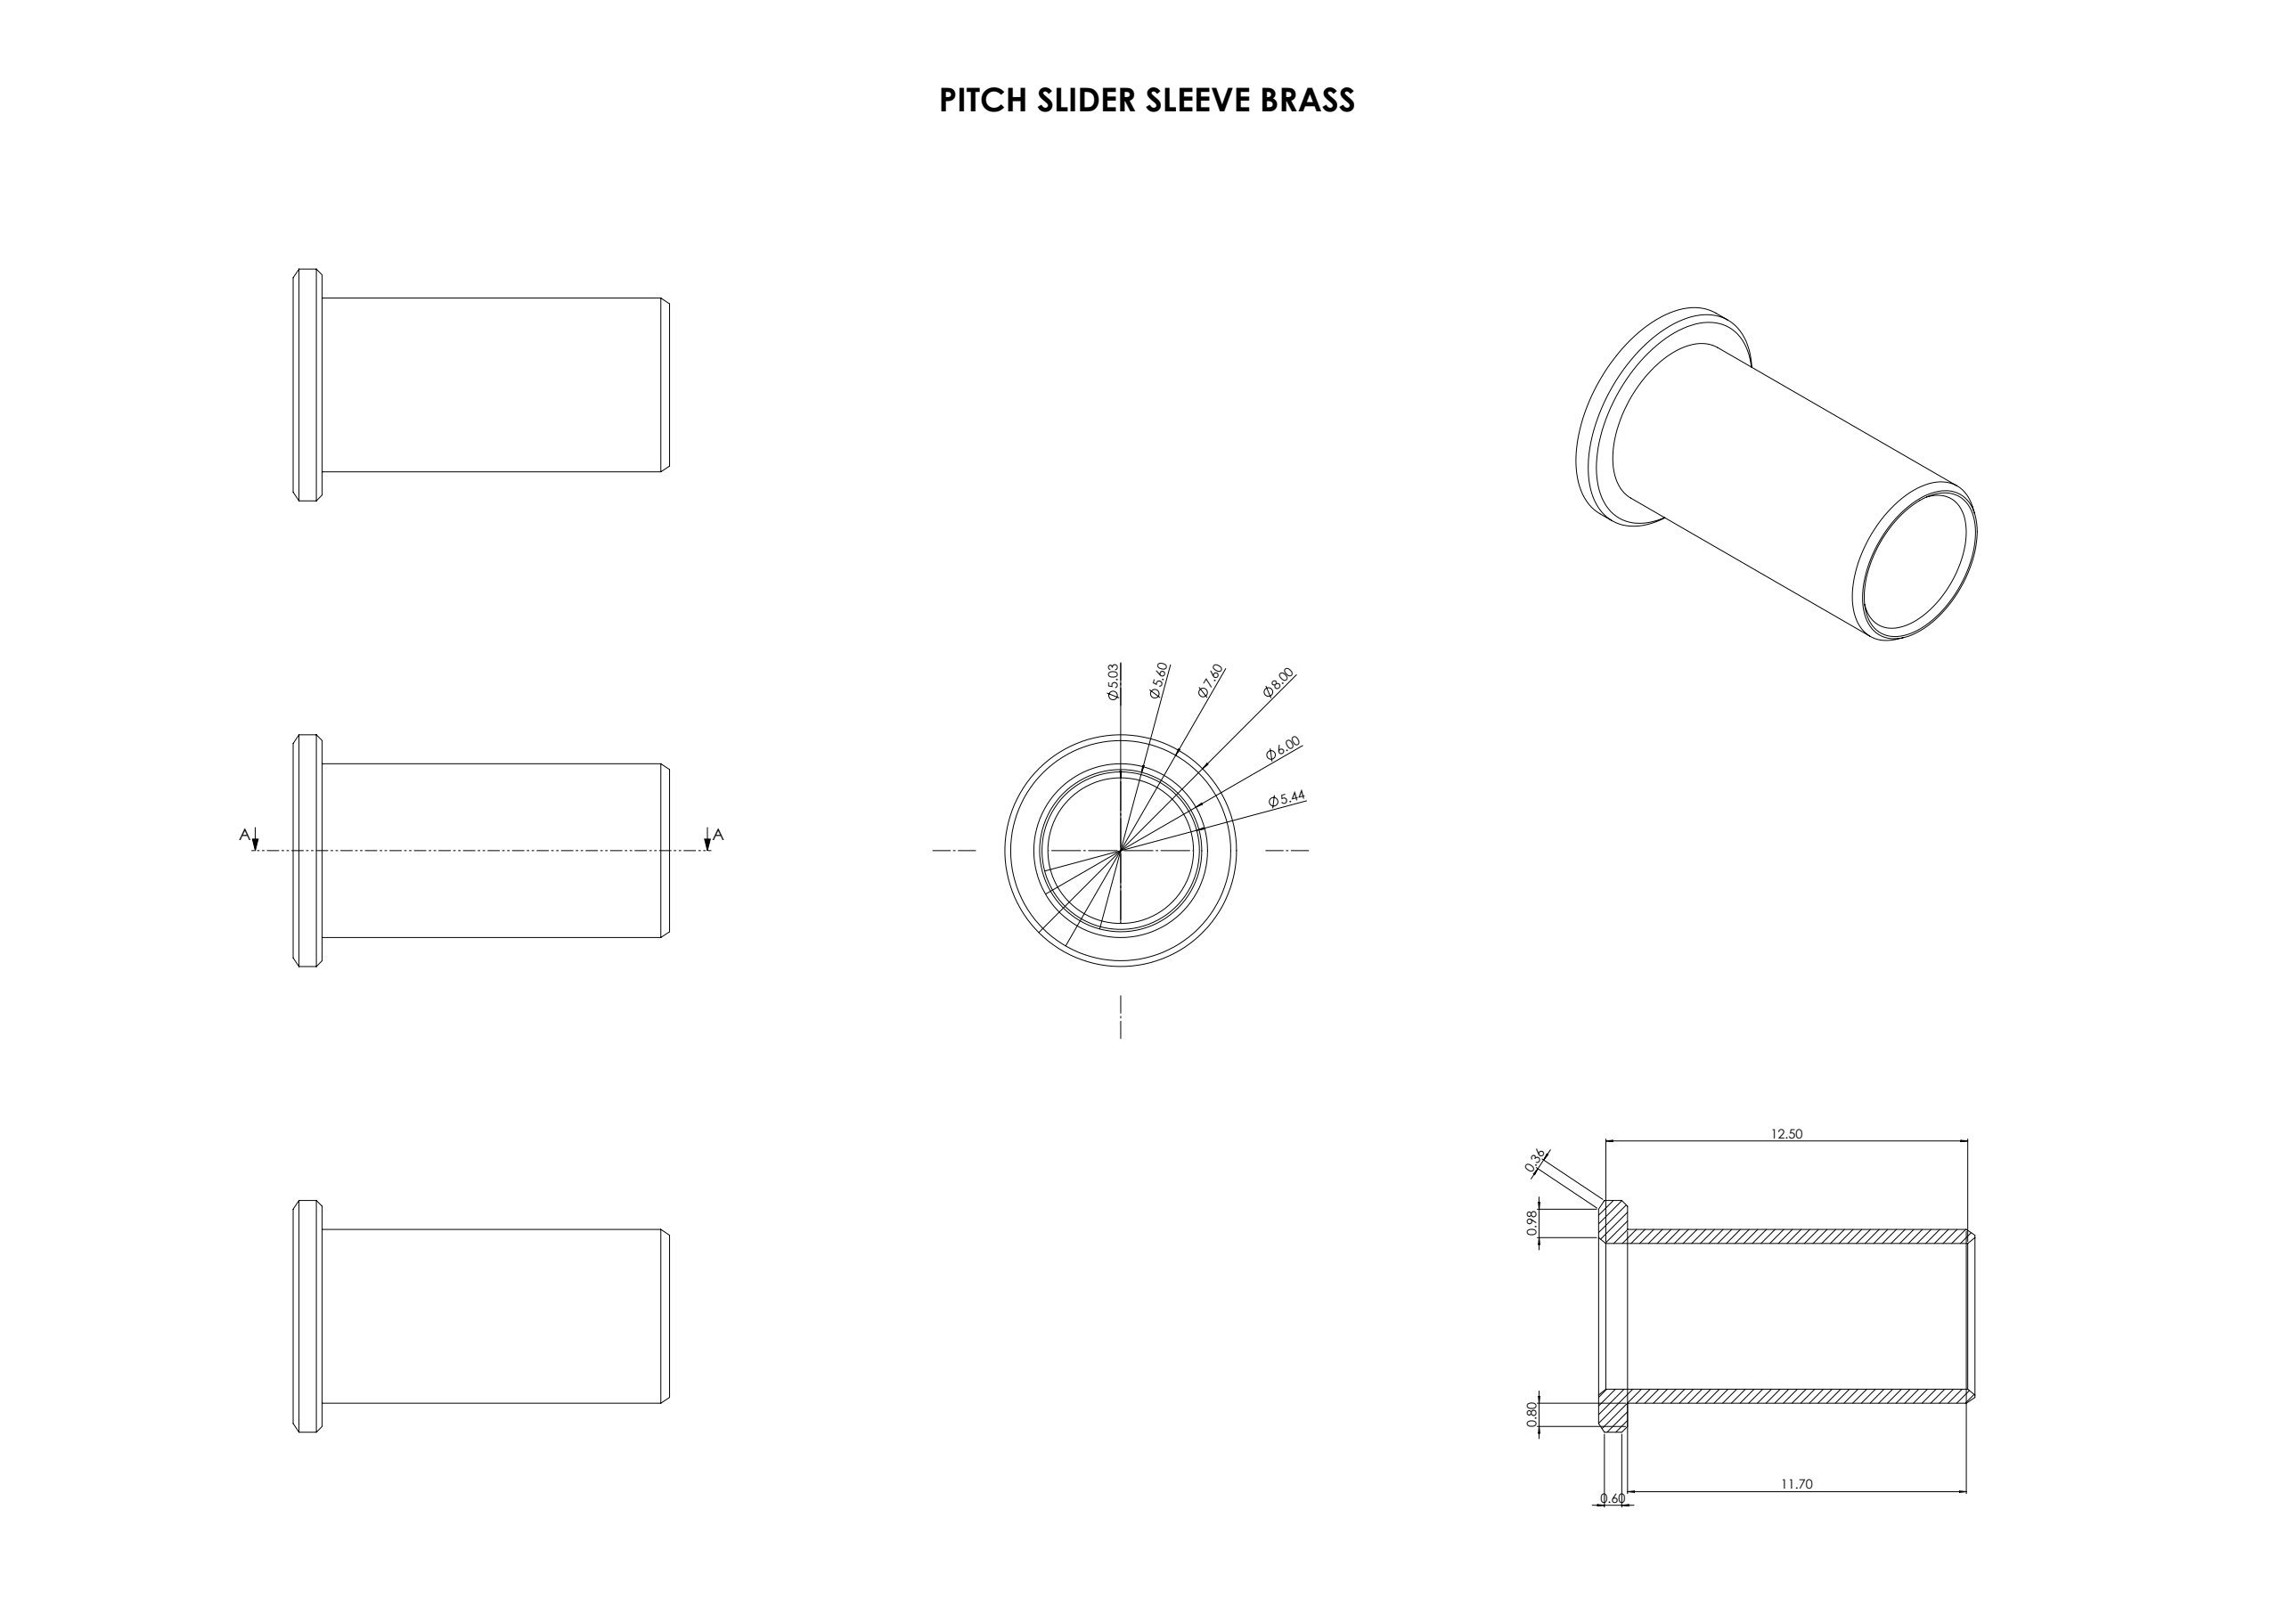
ISO-10303-21;
HEADER;
/* Generated by software containing ST-Developer
 * from STEP Tools, Inc. (www.steptools.com) 
 */

FILE_DESCRIPTION(
/* description */ (''),
/* implementation_level */ '2;1');

FILE_NAME(
/* name */ '02_Pitch_Slider_Sleeve_Brass.step',
/* time_stamp */ '2026-10-25T01:35:35-07:00',
/* author */ (''),
/* organization */ (''),
/* preprocessor_version */ 'ST-DEVELOPER v20.2',
/* originating_system */ 'Autodesk Translation Framework v15.15.0.0',
/* authorisation */ '');

FILE_SCHEMA (('AUTOMOTIVE_DESIGN { 1 0 10303 214 3 1 1 }'));
ENDSEC;

DATA;
#10=MECHANICAL_DESIGN_GEOMETRIC_PRESENTATION_REPRESENTATION('',(#261),#11430);
#237=SHAPE_REPRESENTATION_RELATIONSHIP('SRR','None',#11480,#249);
#249=ADVANCED_BREP_SHAPE_REPRESENTATION('',(#273),#11419);
#261=STYLED_ITEM('',(#11602),#273);
#273=MANIFOLD_SOLID_BREP('Body1',#4462);
#289=FACE_BOUND('',#842,.T.);
#290=FACE_BOUND('',#847,.T.);
#291=FACE_BOUND('',#851,.T.);
#342=PLANE('',#4685);
#343=PLANE('',#4693);
#344=PLANE('',#4699);
#440=CYLINDRICAL_SURFACE('',#4684,2.515);
#441=CYLINDRICAL_SURFACE('',#4689,4.);
#442=CYLINDRICAL_SURFACE('',#4695,3.);
#565=FACE_OUTER_BOUND('',#838,.T.);
#566=FACE_OUTER_BOUND('',#839,.T.);
#567=FACE_OUTER_BOUND('',#840,.T.);
#568=FACE_OUTER_BOUND('',#841,.T.);
#569=FACE_OUTER_BOUND('',#843,.T.);
#570=FACE_OUTER_BOUND('',#844,.T.);
#571=FACE_OUTER_BOUND('',#845,.T.);
#572=FACE_OUTER_BOUND('',#846,.T.);
#573=FACE_OUTER_BOUND('',#848,.T.);
#574=FACE_OUTER_BOUND('',#849,.T.);
#575=FACE_OUTER_BOUND('',#850,.T.);
#838=EDGE_LOOP('',(#3045,#3046,#3047,#3048));
#839=EDGE_LOOP('',(#3049,#3050,#3051,#3052));
#840=EDGE_LOOP('',(#3053,#3054,#3055,#3056));
#841=EDGE_LOOP('',(#3057));
#842=EDGE_LOOP('',(#3058));
#843=EDGE_LOOP('',(#3059,#3060,#3061,#3062));
#844=EDGE_LOOP('',(#3063,#3064,#3065,#3066));
#845=EDGE_LOOP('',(#3067,#3068,#3069,#3070));
#846=EDGE_LOOP('',(#3071));
#847=EDGE_LOOP('',(#3072));
#848=EDGE_LOOP('',(#3073,#3074,#3075,#3076));
#849=EDGE_LOOP('',(#3077,#3078,#3079,#3080));
#850=EDGE_LOOP('',(#3081));
#851=EDGE_LOOP('',(#3082));
#1151=LINE('',#6499,#1441);
#1152=LINE('',#6505,#1442);
#1153=LINE('',#6508,#1443);
#1154=LINE('',#6515,#1444);
#1155=LINE('',#6519,#1445);
#1156=LINE('',#6523,#1446);
#1157=LINE('',#6530,#1447);
#1158=LINE('',#6534,#1448);
#1441=VECTOR('',#5281,2.6575);
#1442=VECTOR('',#5288,2.6575);
#1443=VECTOR('',#5293,2.515);
#1444=VECTOR('',#5302,3.85);
#1445=VECTOR('',#5307,4.);
#1446=VECTOR('',#5312,3.9);
#1447=VECTOR('',#5321,3.);
#1448=VECTOR('',#5326,2.9);
#1711=CIRCLE('',#4679,2.515);
#1712=CIRCLE('',#4680,2.71857142857143);
#1713=CIRCLE('',#4682,2.71857142857143);
#1714=CIRCLE('',#4683,2.515);
#1715=CIRCLE('',#4686,3.7);
#1716=CIRCLE('',#4688,4.);
#1717=CIRCLE('',#4690,4.);
#1718=CIRCLE('',#4692,3.8);
#1719=CIRCLE('',#4694,3.);
#1720=CIRCLE('',#4696,3.);
#1721=CIRCLE('',#4698,2.8);
#1912=VERTEX_POINT('',#6496);
#1913=VERTEX_POINT('',#6498);
#1914=VERTEX_POINT('',#6502);
#1915=VERTEX_POINT('',#6504);
#1916=VERTEX_POINT('',#6510);
#1917=VERTEX_POINT('',#6513);
#1918=VERTEX_POINT('',#6517);
#1919=VERTEX_POINT('',#6521);
#1920=VERTEX_POINT('',#6525);
#1921=VERTEX_POINT('',#6528);
#1922=VERTEX_POINT('',#6532);
#2340=EDGE_CURVE('',#1912,#1912,#1711,.T.);
#2341=EDGE_CURVE('',#1912,#1913,#1151,.T.);
#2342=EDGE_CURVE('',#1913,#1913,#1712,.T.);
#2343=EDGE_CURVE('',#1914,#1914,#1713,.T.);
#2344=EDGE_CURVE('',#1914,#1915,#1152,.T.);
#2345=EDGE_CURVE('',#1915,#1915,#1714,.T.);
#2346=EDGE_CURVE('',#1912,#1915,#1153,.T.);
#2347=EDGE_CURVE('',#1916,#1916,#1715,.T.);
#2348=EDGE_CURVE('',#1917,#1917,#1716,.T.);
#2349=EDGE_CURVE('',#1917,#1916,#1154,.T.);
#2350=EDGE_CURVE('',#1918,#1918,#1717,.T.);
#2351=EDGE_CURVE('',#1918,#1917,#1155,.T.);
#2352=EDGE_CURVE('',#1919,#1919,#1718,.T.);
#2353=EDGE_CURVE('',#1919,#1918,#1156,.T.);
#2354=EDGE_CURVE('',#1920,#1920,#1719,.T.);
#2355=EDGE_CURVE('',#1921,#1921,#1720,.T.);
#2356=EDGE_CURVE('',#1921,#1920,#1157,.T.);
#2357=EDGE_CURVE('',#1922,#1922,#1721,.T.);
#2358=EDGE_CURVE('',#1922,#1921,#1158,.T.);
#3045=ORIENTED_EDGE('',*,*,#2340,.F.);
#3046=ORIENTED_EDGE('',*,*,#2341,.T.);
#3047=ORIENTED_EDGE('',*,*,#2342,.F.);
#3048=ORIENTED_EDGE('',*,*,#2341,.F.);
#3049=ORIENTED_EDGE('',*,*,#2343,.F.);
#3050=ORIENTED_EDGE('',*,*,#2344,.T.);
#3051=ORIENTED_EDGE('',*,*,#2345,.F.);
#3052=ORIENTED_EDGE('',*,*,#2344,.F.);
#3053=ORIENTED_EDGE('',*,*,#2340,.T.);
#3054=ORIENTED_EDGE('',*,*,#2346,.T.);
#3055=ORIENTED_EDGE('',*,*,#2345,.T.);
#3056=ORIENTED_EDGE('',*,*,#2346,.F.);
#3057=ORIENTED_EDGE('',*,*,#2347,.F.);
#3058=ORIENTED_EDGE('',*,*,#2343,.T.);
#3059=ORIENTED_EDGE('',*,*,#2348,.F.);
#3060=ORIENTED_EDGE('',*,*,#2349,.T.);
#3061=ORIENTED_EDGE('',*,*,#2347,.T.);
#3062=ORIENTED_EDGE('',*,*,#2349,.F.);
#3063=ORIENTED_EDGE('',*,*,#2350,.F.);
#3064=ORIENTED_EDGE('',*,*,#2351,.T.);
#3065=ORIENTED_EDGE('',*,*,#2348,.T.);
#3066=ORIENTED_EDGE('',*,*,#2351,.F.);
#3067=ORIENTED_EDGE('',*,*,#2352,.F.);
#3068=ORIENTED_EDGE('',*,*,#2353,.T.);
#3069=ORIENTED_EDGE('',*,*,#2350,.T.);
#3070=ORIENTED_EDGE('',*,*,#2353,.F.);
#3071=ORIENTED_EDGE('',*,*,#2352,.T.);
#3072=ORIENTED_EDGE('',*,*,#2354,.F.);
#3073=ORIENTED_EDGE('',*,*,#2355,.F.);
#3074=ORIENTED_EDGE('',*,*,#2356,.T.);
#3075=ORIENTED_EDGE('',*,*,#2354,.T.);
#3076=ORIENTED_EDGE('',*,*,#2356,.F.);
#3077=ORIENTED_EDGE('',*,*,#2357,.F.);
#3078=ORIENTED_EDGE('',*,*,#2358,.T.);
#3079=ORIENTED_EDGE('',*,*,#2355,.T.);
#3080=ORIENTED_EDGE('',*,*,#2358,.F.);
#3081=ORIENTED_EDGE('',*,*,#2357,.T.);
#3082=ORIENTED_EDGE('',*,*,#2342,.T.);
#4146=CONICAL_SURFACE('',#4678,2.6575,0.683391245487337);
#4147=CONICAL_SURFACE('',#4681,2.6575,0.683391245487336);
#4148=CONICAL_SURFACE('',#4687,3.85,0.982793723247329);
#4149=CONICAL_SURFACE('',#4691,3.9,0.785398163397449);
#4150=CONICAL_SURFACE('',#4697,2.9,0.588002603547568);
#4232=ADVANCED_FACE('',(#565),#4146,.F.);
#4233=ADVANCED_FACE('',(#566),#4147,.F.);
#4234=ADVANCED_FACE('',(#567),#440,.F.);
#4235=ADVANCED_FACE('',(#568,#289),#342,.T.);
#4236=ADVANCED_FACE('',(#569),#4148,.T.);
#4237=ADVANCED_FACE('',(#570),#441,.T.);
#4238=ADVANCED_FACE('',(#571),#4149,.T.);
#4239=ADVANCED_FACE('',(#572,#290),#343,.T.);
#4240=ADVANCED_FACE('',(#573),#442,.T.);
#4241=ADVANCED_FACE('',(#574),#4150,.T.);
#4242=ADVANCED_FACE('',(#575,#291),#344,.T.);
#4462=CLOSED_SHELL('',(#4232,#4233,#4234,#4235,#4236,#4237,#4238,#4239,
#4240,#4241,#4242));
#4677=AXIS2_PLACEMENT_3D('',#6494,#5275,#5276);
#4678=AXIS2_PLACEMENT_3D('',#6495,#5277,#5278);
#4679=AXIS2_PLACEMENT_3D('',#6497,#5279,#5280);
#4680=AXIS2_PLACEMENT_3D('',#6500,#5282,#5283);
#4681=AXIS2_PLACEMENT_3D('',#6501,#5284,#5285);
#4682=AXIS2_PLACEMENT_3D('',#6503,#5286,#5287);
#4683=AXIS2_PLACEMENT_3D('',#6506,#5289,#5290);
#4684=AXIS2_PLACEMENT_3D('',#6507,#5291,#5292);
#4685=AXIS2_PLACEMENT_3D('',#6509,#5294,#5295);
#4686=AXIS2_PLACEMENT_3D('',#6511,#5296,#5297);
#4687=AXIS2_PLACEMENT_3D('',#6512,#5298,#5299);
#4688=AXIS2_PLACEMENT_3D('',#6514,#5300,#5301);
#4689=AXIS2_PLACEMENT_3D('',#6516,#5303,#5304);
#4690=AXIS2_PLACEMENT_3D('',#6518,#5305,#5306);
#4691=AXIS2_PLACEMENT_3D('',#6520,#5308,#5309);
#4692=AXIS2_PLACEMENT_3D('',#6522,#5310,#5311);
#4693=AXIS2_PLACEMENT_3D('',#6524,#5313,#5314);
#4694=AXIS2_PLACEMENT_3D('',#6526,#5315,#5316);
#4695=AXIS2_PLACEMENT_3D('',#6527,#5317,#5318);
#4696=AXIS2_PLACEMENT_3D('',#6529,#5319,#5320);
#4697=AXIS2_PLACEMENT_3D('',#6531,#5322,#5323);
#4698=AXIS2_PLACEMENT_3D('',#6533,#5324,#5325);
#4699=AXIS2_PLACEMENT_3D('',#6535,#5327,#5328);
#5275=DIRECTION('axis',(0.,0.,1.));
#5276=DIRECTION('refdir',(1.,0.,0.));
#5277=DIRECTION('center_axis',(1.,0.,0.));
#5278=DIRECTION('ref_axis',(0.,1.,0.));
#5279=DIRECTION('center_axis',(1.,0.,0.));
#5280=DIRECTION('ref_axis',(0.,1.,0.));
#5281=DIRECTION('',(0.775435860081924,-0.631426343209568,-7.73274250108915E-17));
#5282=DIRECTION('center_axis',(-1.,0.,0.));
#5283=DIRECTION('ref_axis',(0.,1.,0.));
#5284=DIRECTION('center_axis',(-1.,0.,0.));
#5285=DIRECTION('ref_axis',(0.,1.,0.));
#5286=DIRECTION('center_axis',(1.,0.,0.));
#5287=DIRECTION('ref_axis',(0.,1.,0.));
#5288=DIRECTION('',(0.775435860081925,0.631426343209567,7.73274250108914E-17));
#5289=DIRECTION('center_axis',(-1.,0.,0.));
#5290=DIRECTION('ref_axis',(0.,1.,0.));
#5291=DIRECTION('center_axis',(1.,0.,0.));
#5292=DIRECTION('ref_axis',(0.,1.,0.));
#5293=DIRECTION('',(-1.,0.,0.));
#5294=DIRECTION('center_axis',(-1.,0.,0.));
#5295=DIRECTION('ref_axis',(0.,0.,1.));
#5296=DIRECTION('center_axis',(1.,0.,0.));
#5297=DIRECTION('ref_axis',(0.,0.,-1.));
#5298=DIRECTION('center_axis',(1.,0.,0.));
#5299=DIRECTION('ref_axis',(0.,1.,0.));
#5300=DIRECTION('center_axis',(1.,0.,0.));
#5301=DIRECTION('ref_axis',(0.,0.,-1.));
#5302=DIRECTION('',(-0.554700196225229,0.832050294337844,1.01896772969045E-16));
#5303=DIRECTION('center_axis',(1.,0.,0.));
#5304=DIRECTION('ref_axis',(0.,1.,0.));
#5305=DIRECTION('center_axis',(1.,0.,0.));
#5306=DIRECTION('ref_axis',(0.,0.,-1.));
#5307=DIRECTION('',(-1.,0.,0.));
#5308=DIRECTION('center_axis',(-1.,0.,0.));
#5309=DIRECTION('ref_axis',(0.,1.,0.));
#5310=DIRECTION('center_axis',(1.,0.,0.));
#5311=DIRECTION('ref_axis',(0.,0.,-1.));
#5312=DIRECTION('',(-0.707106781186547,-0.707106781186548,-8.65956056235494E-17));
#5313=DIRECTION('center_axis',(1.,0.,0.));
#5314=DIRECTION('ref_axis',(0.,0.,-1.));
#5315=DIRECTION('center_axis',(1.,0.,0.));
#5316=DIRECTION('ref_axis',(0.,0.,-1.));
#5317=DIRECTION('center_axis',(1.,0.,0.));
#5318=DIRECTION('ref_axis',(0.,1.,0.));
#5319=DIRECTION('center_axis',(1.,0.,0.));
#5320=DIRECTION('ref_axis',(0.,0.,-1.));
#5321=DIRECTION('',(-1.,0.,0.));
#5322=DIRECTION('center_axis',(-1.,0.,0.));
#5323=DIRECTION('ref_axis',(0.,1.,0.));
#5324=DIRECTION('center_axis',(1.,0.,0.));
#5325=DIRECTION('ref_axis',(0.,0.,-1.));
#5326=DIRECTION('',(-0.832050294337844,-0.554700196225229,-6.79311819793636E-17));
#5327=DIRECTION('center_axis',(1.,0.,0.));
#5328=DIRECTION('ref_axis',(0.,0.,-1.));
#6494=CARTESIAN_POINT('',(0.,0.,0.));
#6495=CARTESIAN_POINT('Origin',(11.925,0.,0.));
#6496=CARTESIAN_POINT('',(11.75,-2.515,-3.07998669985559E-16));
#6497=CARTESIAN_POINT('Origin',(11.75,0.,0.));
#6498=CARTESIAN_POINT('',(12.,-2.71857142857143,3.32928979825345E-16));
#6499=CARTESIAN_POINT('',(11.925,-2.6575,-3.25449886873409E-16));
#6500=CARTESIAN_POINT('Origin',(12.,0.,0.));
#6501=CARTESIAN_POINT('Origin',(-0.925,0.,0.));
#6502=CARTESIAN_POINT('',(-1.,-2.71857142857143,-3.32928979825345E-16));
#6503=CARTESIAN_POINT('Origin',(-1.,0.,0.));
#6504=CARTESIAN_POINT('',(-0.75,-2.515,-3.07998669985559E-16));
#6505=CARTESIAN_POINT('',(-0.925,-2.6575,-3.25449886873409E-16));
#6506=CARTESIAN_POINT('Origin',(-0.750000000000001,0.,0.));
#6507=CARTESIAN_POINT('Origin',(5.5,0.,0.));
#6508=CARTESIAN_POINT('',(5.5,-2.515,-3.07998669985559E-16));
#6509=CARTESIAN_POINT('Origin',(-1.,3.7,0.));
#6510=CARTESIAN_POINT('',(-1.,-3.7,-4.53119315684521E-16));
#6511=CARTESIAN_POINT('Origin',(-1.,0.,0.));
#6512=CARTESIAN_POINT('Origin',(-0.900000000000001,0.,0.));
#6513=CARTESIAN_POINT('',(-0.800000000000001,-4.,-4.89858719658941E-16));
#6514=CARTESIAN_POINT('Origin',(-0.800000000000001,0.,0.));
#6515=CARTESIAN_POINT('',(-0.900000000000001,-3.85,-4.71489017671731E-16));
#6516=CARTESIAN_POINT('Origin',(-0.5,0.,0.));
#6517=CARTESIAN_POINT('',(-0.2,-4.,-4.89858719658941E-16));
#6518=CARTESIAN_POINT('Origin',(-0.2,0.,0.));
#6519=CARTESIAN_POINT('',(-0.5,-4.,-4.89858719658941E-16));
#6520=CARTESIAN_POINT('Origin',(-0.1,0.,0.));
#6521=CARTESIAN_POINT('',(1.73472347597681E-17,-3.8,-4.65365783675994E-16));
#6522=CARTESIAN_POINT('Origin',(0.,0.,0.));
#6523=CARTESIAN_POINT('',(-0.1,-3.9,-4.77612251667468E-16));
#6524=CARTESIAN_POINT('Origin',(0.,3.,0.));
#6525=CARTESIAN_POINT('',(0.,-3.,-3.67394039744206E-16));
#6526=CARTESIAN_POINT('Origin',(0.,0.,0.));
#6527=CARTESIAN_POINT('Origin',(5.85,0.,0.));
#6528=CARTESIAN_POINT('',(11.7,-3.,-3.67394039744206E-16));
#6529=CARTESIAN_POINT('Origin',(11.7,0.,0.));
#6530=CARTESIAN_POINT('',(5.85,-3.,-3.67394039744206E-16));
#6531=CARTESIAN_POINT('Origin',(11.85,0.,0.));
#6532=CARTESIAN_POINT('',(12.,-2.8,-3.42901103761259E-16));
#6533=CARTESIAN_POINT('Origin',(12.,0.,0.));
#6534=CARTESIAN_POINT('',(11.85,-2.9,-3.55147571752732E-16));
#6535=CARTESIAN_POINT('Origin',(12.,2.515,0.));
#11405=UNCERTAINTY_MEASURE_WITH_UNIT(LENGTH_MEASURE(0.01),#11431,
'DISTANCE_ACCURACY_VALUE',
'Maximum model space distance between geometric entities at asserted c
onnectivities');
#11416=UNCERTAINTY_MEASURE_WITH_UNIT(LENGTH_MEASURE(0.01),#11431,
'DISTANCE_ACCURACY_VALUE',
'Maximum model space distance between geometric entities at asserted c
onnectivities');
#11419=(
GEOMETRIC_REPRESENTATION_CONTEXT(3)
GLOBAL_UNCERTAINTY_ASSIGNED_CONTEXT((#11405))
GLOBAL_UNIT_ASSIGNED_CONTEXT((#11431,#11433,#11434))
REPRESENTATION_CONTEXT('','3D')
);
#11430=(
GEOMETRIC_REPRESENTATION_CONTEXT(3)
GLOBAL_UNCERTAINTY_ASSIGNED_CONTEXT((#11416))
GLOBAL_UNIT_ASSIGNED_CONTEXT((#11431,#11433,#11434))
REPRESENTATION_CONTEXT('','3D')
);
#11431=(
LENGTH_UNIT()
NAMED_UNIT(*)
SI_UNIT(.MILLI.,.METRE.)
);
#11433=(
NAMED_UNIT(*)
PLANE_ANGLE_UNIT()
SI_UNIT($,.RADIAN.)
);
#11434=(
NAMED_UNIT(*)
SI_UNIT($,.STERADIAN.)
SOLID_ANGLE_UNIT()
);
#11437=SHAPE_DEFINITION_REPRESENTATION(#11450,#11480);
#11450=PRODUCT_DEFINITION_SHAPE('',$,#11494);
#11480=SHAPE_REPRESENTATION('',(#4677),#11419);
#11491=PRODUCT_DEFINITION_CONTEXT('part definition',#11532,'design');
#11494=PRODUCT_DEFINITION('2026-10-25-00-55-37-452',
'02_Pitch_Slider_Sleeve_Brass',#11507,#11491);
#11507=PRODUCT_DEFINITION_FORMATION('',$,#11536);
#11532=APPLICATION_CONTEXT(
'Core Data for Automotive Mechanical Design Process');
#11533=PRODUCT_CONTEXT('part definition',#11532,'mechanical');
#11536=PRODUCT('2026-10-25-00-55-37-452','02_Pitch_Slider_Sleeve_Brass',
$,(#11533));
#11596=COLOUR_RGB('Sky Blue',0.24,0.69,0.87);
#11597=FILL_AREA_STYLE_COLOUR('',#11596);
#11598=FILL_AREA_STYLE('',(#11597));
#11599=SURFACE_STYLE_FILL_AREA(#11598);
#11600=SURFACE_SIDE_STYLE('',(#11599));
#11601=SURFACE_STYLE_USAGE(.BOTH.,#11600);
#11602=PRESENTATION_STYLE_ASSIGNMENT((#11601));
ENDSEC;
END-ISO-10303-21;
